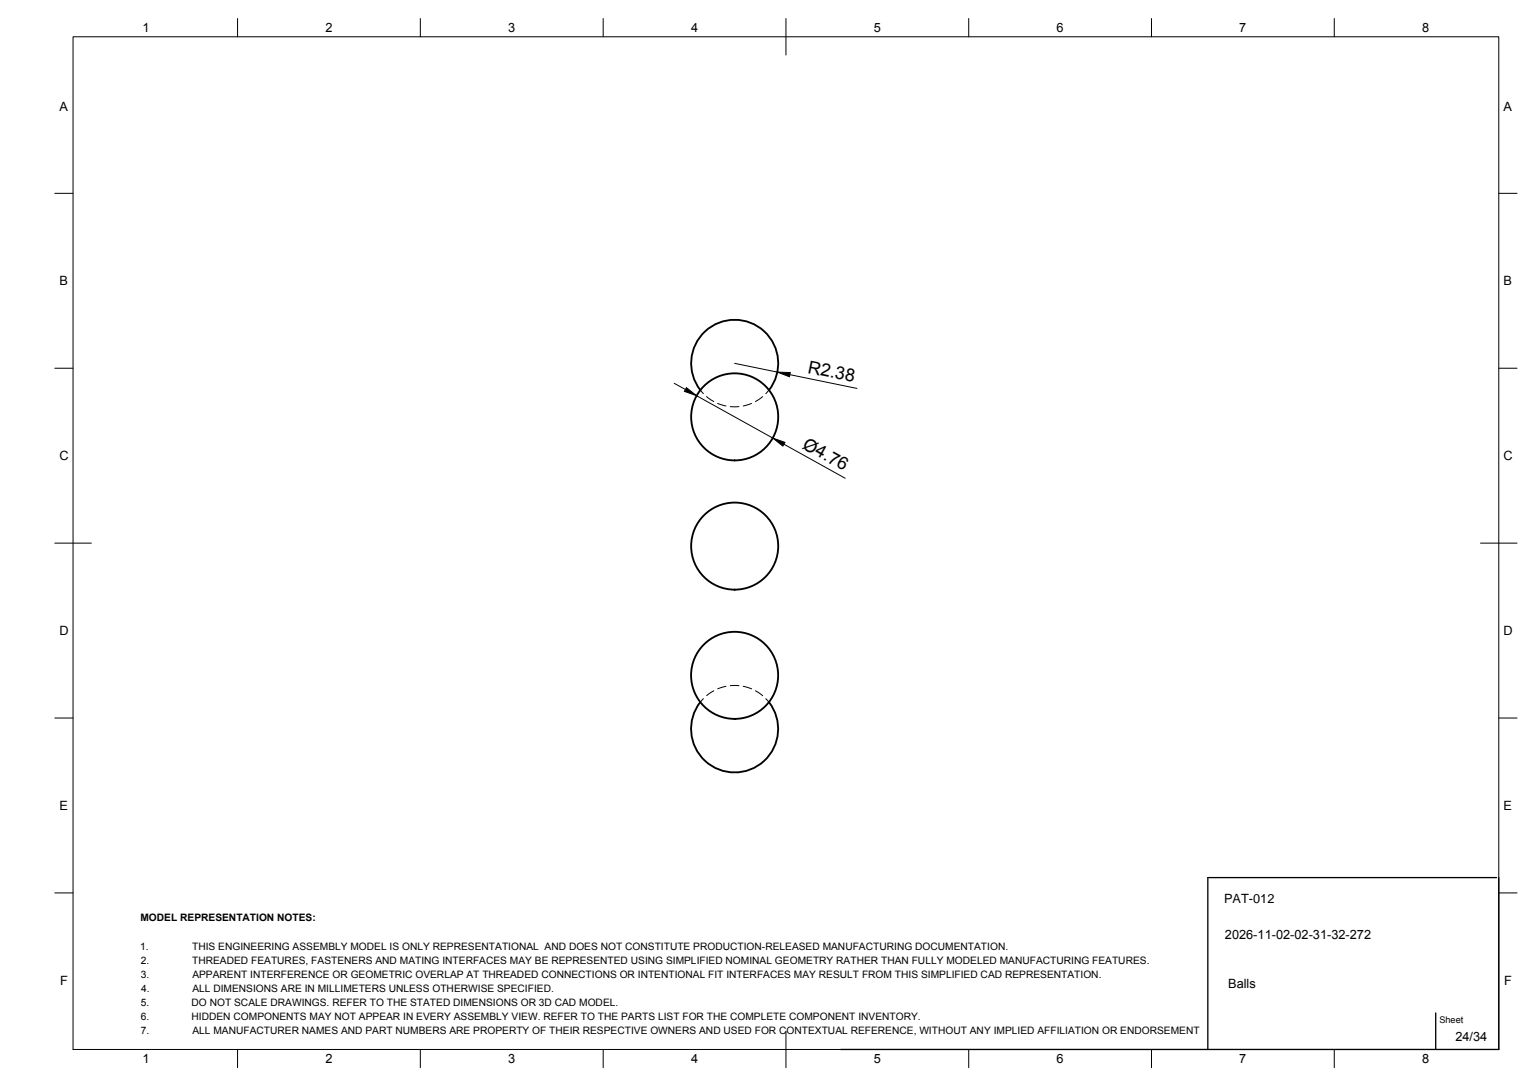
ISO-10303-21;
HEADER;
/* Generated by software containing ST-Developer
 * from STEP Tools, Inc. (www.steptools.com) 
 */

FILE_DESCRIPTION(
/* description */ ('Belt tensioner idler arm'),
/* implementation_level */ '2;1');

FILE_NAME(
/* name */ 'Balls.step',
/* time_stamp */ '2026-10-28T03:22:15-07:00',
/* author */ (''),
/* organization */ (''),
/* preprocessor_version */ 'ST-DEVELOPER v20.2',
/* originating_system */ 'Autodesk Translation Framework v15.17.0.0',
/* authorisation */ '');

FILE_SCHEMA (('AUTOMOTIVE_DESIGN { 1 0 10303 214 3 1 1 }'));
ENDSEC;

DATA;
#10=MECHANICAL_DESIGN_GEOMETRIC_PRESENTATION_REPRESENTATION('',(#467,#468,#469,#470,#471,#472,#473,#474),#12779);
#255=SPHERICAL_SURFACE('',#7008,0.23815);
#256=SPHERICAL_SURFACE('',#7010,0.23815);
#257=SPHERICAL_SURFACE('',#7012,0.23815);
#258=SPHERICAL_SURFACE('',#7014,0.23815);
#259=SPHERICAL_SURFACE('',#7016,0.23815);
#260=SPHERICAL_SURFACE('',#7018,0.23815);
#261=SPHERICAL_SURFACE('',#7020,0.23815);
#262=SPHERICAL_SURFACE('',#7022,0.23815);
#399=SHAPE_REPRESENTATION_RELATIONSHIP('SRR','None',#12947,#433);
#433=ADVANCED_BREP_SHAPE_REPRESENTATION('',(#507,#508,#509,#510,#511,#512,
#513,#514),#12764);
#467=STYLED_ITEM('',(#13184),#507);
#468=STYLED_ITEM('',(#13184),#508);
#469=STYLED_ITEM('',(#13184),#509);
#470=STYLED_ITEM('',(#13184),#510);
#471=STYLED_ITEM('',(#13184),#511);
#472=STYLED_ITEM('',(#13184),#512);
#473=STYLED_ITEM('',(#13184),#513);
#474=STYLED_ITEM('',(#13184),#514);
#507=MANIFOLD_SOLID_BREP('Body1',#6203);
#508=MANIFOLD_SOLID_BREP('Body2',#6204);
#509=MANIFOLD_SOLID_BREP('Body3',#6205);
#510=MANIFOLD_SOLID_BREP('Body4',#6206);
#511=MANIFOLD_SOLID_BREP('Body5',#6207);
#512=MANIFOLD_SOLID_BREP('Body6',#6208);
#513=MANIFOLD_SOLID_BREP('Body7',#6209);
#514=MANIFOLD_SOLID_BREP('Body8',#6210);
#1039=FACE_OUTER_BOUND('',#1510,.T.);
#1040=FACE_OUTER_BOUND('',#1511,.T.);
#1041=FACE_OUTER_BOUND('',#1512,.T.);
#1042=FACE_OUTER_BOUND('',#1513,.T.);
#1043=FACE_OUTER_BOUND('',#1514,.T.);
#1044=FACE_OUTER_BOUND('',#1515,.T.);
#1045=FACE_OUTER_BOUND('',#1516,.T.);
#1046=FACE_OUTER_BOUND('',#1517,.T.);
#1510=EDGE_LOOP('',(#4924,#4925));
#1511=EDGE_LOOP('',(#4926,#4927));
#1512=EDGE_LOOP('',(#4928,#4929));
#1513=EDGE_LOOP('',(#4930,#4931));
#1514=EDGE_LOOP('',(#4932,#4933));
#1515=EDGE_LOOP('',(#4934,#4935));
#1516=EDGE_LOOP('',(#4936,#4937));
#1517=EDGE_LOOP('',(#4938,#4939));
#2584=CIRCLE('',#7009,0.23815);
#2585=CIRCLE('',#7011,0.23815);
#2586=CIRCLE('',#7013,0.23815);
#2587=CIRCLE('',#7015,0.23815);
#2588=CIRCLE('',#7017,0.23815);
#2589=CIRCLE('',#7019,0.23815);
#2590=CIRCLE('',#7021,0.23815);
#2591=CIRCLE('',#7023,0.23815);
#3040=VERTEX_POINT('',#11157);
#3041=VERTEX_POINT('',#11158);
#3042=VERTEX_POINT('',#11161);
#3043=VERTEX_POINT('',#11162);
#3044=VERTEX_POINT('',#11165);
#3045=VERTEX_POINT('',#11166);
#3046=VERTEX_POINT('',#11169);
#3047=VERTEX_POINT('',#11170);
#3048=VERTEX_POINT('',#11173);
#3049=VERTEX_POINT('',#11174);
#3050=VERTEX_POINT('',#11177);
#3051=VERTEX_POINT('',#11178);
#3052=VERTEX_POINT('',#11181);
#3053=VERTEX_POINT('',#11182);
#3054=VERTEX_POINT('',#11185);
#3055=VERTEX_POINT('',#11186);
#3717=EDGE_CURVE('',#3040,#3041,#2584,.T.);
#3718=EDGE_CURVE('',#3042,#3043,#2585,.T.);
#3719=EDGE_CURVE('',#3044,#3045,#2586,.T.);
#3720=EDGE_CURVE('',#3046,#3047,#2587,.T.);
#3721=EDGE_CURVE('',#3048,#3049,#2588,.T.);
#3722=EDGE_CURVE('',#3050,#3051,#2589,.T.);
#3723=EDGE_CURVE('',#3052,#3053,#2590,.T.);
#3724=EDGE_CURVE('',#3054,#3055,#2591,.T.);
#4924=ORIENTED_EDGE('',*,*,#3717,.T.);
#4925=ORIENTED_EDGE('',*,*,#3717,.F.);
#4926=ORIENTED_EDGE('',*,*,#3718,.T.);
#4927=ORIENTED_EDGE('',*,*,#3718,.F.);
#4928=ORIENTED_EDGE('',*,*,#3719,.T.);
#4929=ORIENTED_EDGE('',*,*,#3719,.F.);
#4930=ORIENTED_EDGE('',*,*,#3720,.T.);
#4931=ORIENTED_EDGE('',*,*,#3720,.F.);
#4932=ORIENTED_EDGE('',*,*,#3721,.T.);
#4933=ORIENTED_EDGE('',*,*,#3721,.F.);
#4934=ORIENTED_EDGE('',*,*,#3722,.T.);
#4935=ORIENTED_EDGE('',*,*,#3722,.F.);
#4936=ORIENTED_EDGE('',*,*,#3723,.T.);
#4937=ORIENTED_EDGE('',*,*,#3723,.F.);
#4938=ORIENTED_EDGE('',*,*,#3724,.T.);
#4939=ORIENTED_EDGE('',*,*,#3724,.F.);
#6016=ADVANCED_FACE('',(#1039),#255,.T.);
#6017=ADVANCED_FACE('',(#1040),#256,.T.);
#6018=ADVANCED_FACE('',(#1041),#257,.T.);
#6019=ADVANCED_FACE('',(#1042),#258,.T.);
#6020=ADVANCED_FACE('',(#1043),#259,.T.);
#6021=ADVANCED_FACE('',(#1044),#260,.T.);
#6022=ADVANCED_FACE('',(#1045),#261,.T.);
#6023=ADVANCED_FACE('',(#1046),#262,.T.);
#6203=CLOSED_SHELL('',(#6016));
#6204=CLOSED_SHELL('',(#6017));
#6205=CLOSED_SHELL('',(#6018));
#6206=CLOSED_SHELL('',(#6019));
#6207=CLOSED_SHELL('',(#6020));
#6208=CLOSED_SHELL('',(#6021));
#6209=CLOSED_SHELL('',(#6022));
#6210=CLOSED_SHELL('',(#6023));
#7007=AXIS2_PLACEMENT_3D('',#11155,#8453,#8454);
#7008=AXIS2_PLACEMENT_3D('',#11156,#8455,#8456);
#7009=AXIS2_PLACEMENT_3D('',#11159,#8457,#8458);
#7010=AXIS2_PLACEMENT_3D('',#11160,#8459,#8460);
#7011=AXIS2_PLACEMENT_3D('',#11163,#8461,#8462);
#7012=AXIS2_PLACEMENT_3D('',#11164,#8463,#8464);
#7013=AXIS2_PLACEMENT_3D('',#11167,#8465,#8466);
#7014=AXIS2_PLACEMENT_3D('',#11168,#8467,#8468);
#7015=AXIS2_PLACEMENT_3D('',#11171,#8469,#8470);
#7016=AXIS2_PLACEMENT_3D('',#11172,#8471,#8472);
#7017=AXIS2_PLACEMENT_3D('',#11175,#8473,#8474);
#7018=AXIS2_PLACEMENT_3D('',#11176,#8475,#8476);
#7019=AXIS2_PLACEMENT_3D('',#11179,#8477,#8478);
#7020=AXIS2_PLACEMENT_3D('',#11180,#8479,#8480);
#7021=AXIS2_PLACEMENT_3D('',#11183,#8481,#8482);
#7022=AXIS2_PLACEMENT_3D('',#11184,#8483,#8484);
#7023=AXIS2_PLACEMENT_3D('',#11187,#8485,#8486);
#8453=DIRECTION('axis',(0.,0.,1.));
#8454=DIRECTION('refdir',(1.,0.,0.));
#8455=DIRECTION('center_axis',(0.,0.,1.));
#8456=DIRECTION('ref_axis',(1.,0.,0.));
#8457=DIRECTION('center_axis',(1.22464679914735E-16,-1.,0.));
#8458=DIRECTION('ref_axis',(-1.,-1.22464679914735E-16,0.));
#8459=DIRECTION('center_axis',(0.707106781186548,0.,0.707106781186548));
#8460=DIRECTION('ref_axis',(0.707106781186548,0.,-0.707106781186548));
#8461=DIRECTION('center_axis',(8.65956056235494E-17,-1.,-8.65956056235493E-17));
#8462=DIRECTION('ref_axis',(-0.707106781186547,-1.22464679914735E-16,0.707106781186547));
#8463=DIRECTION('center_axis',(1.,0.,0.));
#8464=DIRECTION('ref_axis',(6.12323399573676E-17,0.,-1.));
#8465=DIRECTION('center_axis',(7.49879891330929E-33,-1.,-1.22464679914735E-16));
#8466=DIRECTION('ref_axis',(-6.12323399573676E-17,-1.22464679914735E-16,
1.));
#8467=DIRECTION('center_axis',(0.707106781186548,0.,-0.707106781186548));
#8468=DIRECTION('ref_axis',(-0.707106781186548,0.,-0.707106781186548));
#8469=DIRECTION('center_axis',(-8.65956056235493E-17,-1.,-8.65956056235494E-17));
#8470=DIRECTION('ref_axis',(0.707106781186547,-1.22464679914735E-16,0.707106781186547));
#8471=DIRECTION('center_axis',(0.,0.,-1.));
#8472=DIRECTION('ref_axis',(-1.,0.,-1.22464679914735E-16));
#8473=DIRECTION('center_axis',(-1.22464679914735E-16,-1.,-1.49975978266186E-32));
#8474=DIRECTION('ref_axis',(1.,-1.22464679914735E-16,1.22464679914735E-16));
#8475=DIRECTION('center_axis',(-0.707106781186547,0.,-0.707106781186548));
#8476=DIRECTION('ref_axis',(-0.707106781186548,0.,0.707106781186547));
#8477=DIRECTION('center_axis',(-8.65956056235493E-17,-1.,8.65956056235493E-17));
#8478=DIRECTION('ref_axis',(0.707106781186548,-1.22464679914735E-16,-0.707106781186547));
#8479=DIRECTION('center_axis',(-1.,0.,0.));
#8480=DIRECTION('ref_axis',(-1.83697019872103E-16,0.,1.));
#8481=DIRECTION('center_axis',(-2.24963967399279E-32,-1.,1.22464679914735E-16));
#8482=DIRECTION('ref_axis',(1.83697019872103E-16,-1.22464679914735E-16,
-1.));
#8483=DIRECTION('center_axis',(-0.707106781186548,0.,0.707106781186548));
#8484=DIRECTION('ref_axis',(0.707106781186547,0.,0.707106781186548));
#8485=DIRECTION('center_axis',(8.65956056235493E-17,-1.,8.65956056235493E-17));
#8486=DIRECTION('ref_axis',(-0.707106781186547,-1.22464679914735E-16,-0.707106781186548));
#11155=CARTESIAN_POINT('',(0.,0.,0.));
#11156=CARTESIAN_POINT('Origin',(1.,0.,0.));
#11157=CARTESIAN_POINT('',(1.,-1.78583896120461E-33,0.23815));
#11158=CARTESIAN_POINT('',(1.,-1.78583896120461E-33,-0.23815));
#11159=CARTESIAN_POINT('Origin',(1.,0.,0.));
#11160=CARTESIAN_POINT('Origin',(0.707106781186548,0.,-0.707106781186547));
#11161=CARTESIAN_POINT('',(0.875504261126124,-1.78583896120461E-33,-0.538709301246971));
#11162=CARTESIAN_POINT('',(0.538709301246971,-1.78583896120461E-33,-0.875504261126124));
#11163=CARTESIAN_POINT('Origin',(0.707106781186548,0.,-0.707106781186547));
#11164=CARTESIAN_POINT('Origin',(6.12323399573677E-17,0.,-1.));
#11165=CARTESIAN_POINT('',(0.23815,-1.78583896120461E-33,-1.));
#11166=CARTESIAN_POINT('',(-0.23815,-1.78583896120461E-33,-1.));
#11167=CARTESIAN_POINT('Origin',(6.12323399573677E-17,0.,-1.));
#11168=CARTESIAN_POINT('Origin',(-0.707106781186547,0.,-0.707106781186548));
#11169=CARTESIAN_POINT('',(-0.538709301246971,-1.78583896120461E-33,-0.875504261126124));
#11170=CARTESIAN_POINT('',(-0.875504261126124,-1.78583896120461E-33,-0.538709301246971));
#11171=CARTESIAN_POINT('Origin',(-0.707106781186547,0.,-0.707106781186548));
#11172=CARTESIAN_POINT('Origin',(-1.,0.,-1.22464679914735E-16));
#11173=CARTESIAN_POINT('',(-1.,-1.78583896120461E-33,-0.23815));
#11174=CARTESIAN_POINT('',(-1.,-1.78583896120461E-33,0.23815));
#11175=CARTESIAN_POINT('Origin',(-1.,0.,-1.22464679914735E-16));
#11176=CARTESIAN_POINT('Origin',(-0.707106781186548,0.,0.707106781186547));
#11177=CARTESIAN_POINT('',(-0.875504261126124,-7.94881478324376E-33,0.538709301246971));
#11178=CARTESIAN_POINT('',(-0.538709301246971,4.37713686083455E-33,0.875504261126124));
#11179=CARTESIAN_POINT('Origin',(-0.707106781186548,0.,0.707106781186547));
#11180=CARTESIAN_POINT('Origin',(-1.83697019872103E-16,0.,1.));
#11181=CARTESIAN_POINT('',(-0.23815,-1.78583896120461E-33,1.));
#11182=CARTESIAN_POINT('',(0.23815,-1.78583896120461E-33,1.));
#11183=CARTESIAN_POINT('Origin',(-1.83697019872103E-16,0.,1.));
#11184=CARTESIAN_POINT('Origin',(0.707106781186547,0.,0.707106781186548));
#11185=CARTESIAN_POINT('',(0.538709301246971,-4.86732687222419E-33,0.875504261126124));
#11186=CARTESIAN_POINT('',(0.875504261126124,1.29564894981497E-33,0.538709301246971));
#11187=CARTESIAN_POINT('Origin',(0.707106781186547,0.,0.707106781186548));
#12724=UNCERTAINTY_MEASURE_WITH_UNIT(LENGTH_MEASURE(0.001),#12780,
'DISTANCE_ACCURACY_VALUE',
'Maximum model space distance between geometric entities at asserted c
onnectivities');
#12739=UNCERTAINTY_MEASURE_WITH_UNIT(LENGTH_MEASURE(0.001),#12780,
'DISTANCE_ACCURACY_VALUE',
'Maximum model space distance between geometric entities at asserted c
onnectivities');
#12764=(
GEOMETRIC_REPRESENTATION_CONTEXT(3)
GLOBAL_UNCERTAINTY_ASSIGNED_CONTEXT((#12724))
GLOBAL_UNIT_ASSIGNED_CONTEXT((#12780,#12782,#12783))
REPRESENTATION_CONTEXT('','3D')
);
#12779=(
GEOMETRIC_REPRESENTATION_CONTEXT(3)
GLOBAL_UNCERTAINTY_ASSIGNED_CONTEXT((#12739))
GLOBAL_UNIT_ASSIGNED_CONTEXT((#12780,#12782,#12783))
REPRESENTATION_CONTEXT('','3D')
);
#12780=(
LENGTH_UNIT()
NAMED_UNIT(*)
SI_UNIT(.CENTI.,.METRE.)
);
#12782=(
NAMED_UNIT(*)
PLANE_ANGLE_UNIT()
SI_UNIT($,.RADIAN.)
);
#12783=(
NAMED_UNIT(*)
SI_UNIT($,.STERADIAN.)
SOLID_ANGLE_UNIT()
);
#12808=SHAPE_DEFINITION_REPRESENTATION(#12847,#12947);
#12847=PRODUCT_DEFINITION_SHAPE('',$,#12987);
#12947=SHAPE_REPRESENTATION('',(#7007),#12764);
#12962=PRODUCT_DEFINITION_CONTEXT('part definition',#13081,'design');
#12987=PRODUCT_DEFINITION('Balls','Balls',#13026,#12962);
#13026=PRODUCT_DEFINITION_FORMATION('',$,#13107);
#13081=APPLICATION_CONTEXT(
'Core Data for Automotive Mechanical Design Process');
#13082=PRODUCT_CONTEXT('part definition',#13081,'mechanical');
#13107=PRODUCT('Balls','Balls','Balls',(#13082));
#13178=COLOUR_RGB('Grey',0.48,0.52,0.57);
#13179=FILL_AREA_STYLE_COLOUR('',#13178);
#13180=FILL_AREA_STYLE('',(#13179));
#13181=SURFACE_STYLE_FILL_AREA(#13180);
#13182=SURFACE_SIDE_STYLE('',(#13181));
#13183=SURFACE_STYLE_USAGE(.BOTH.,#13182);
#13184=PRESENTATION_STYLE_ASSIGNMENT((#13183));
ENDSEC;
END-ISO-10303-21;
